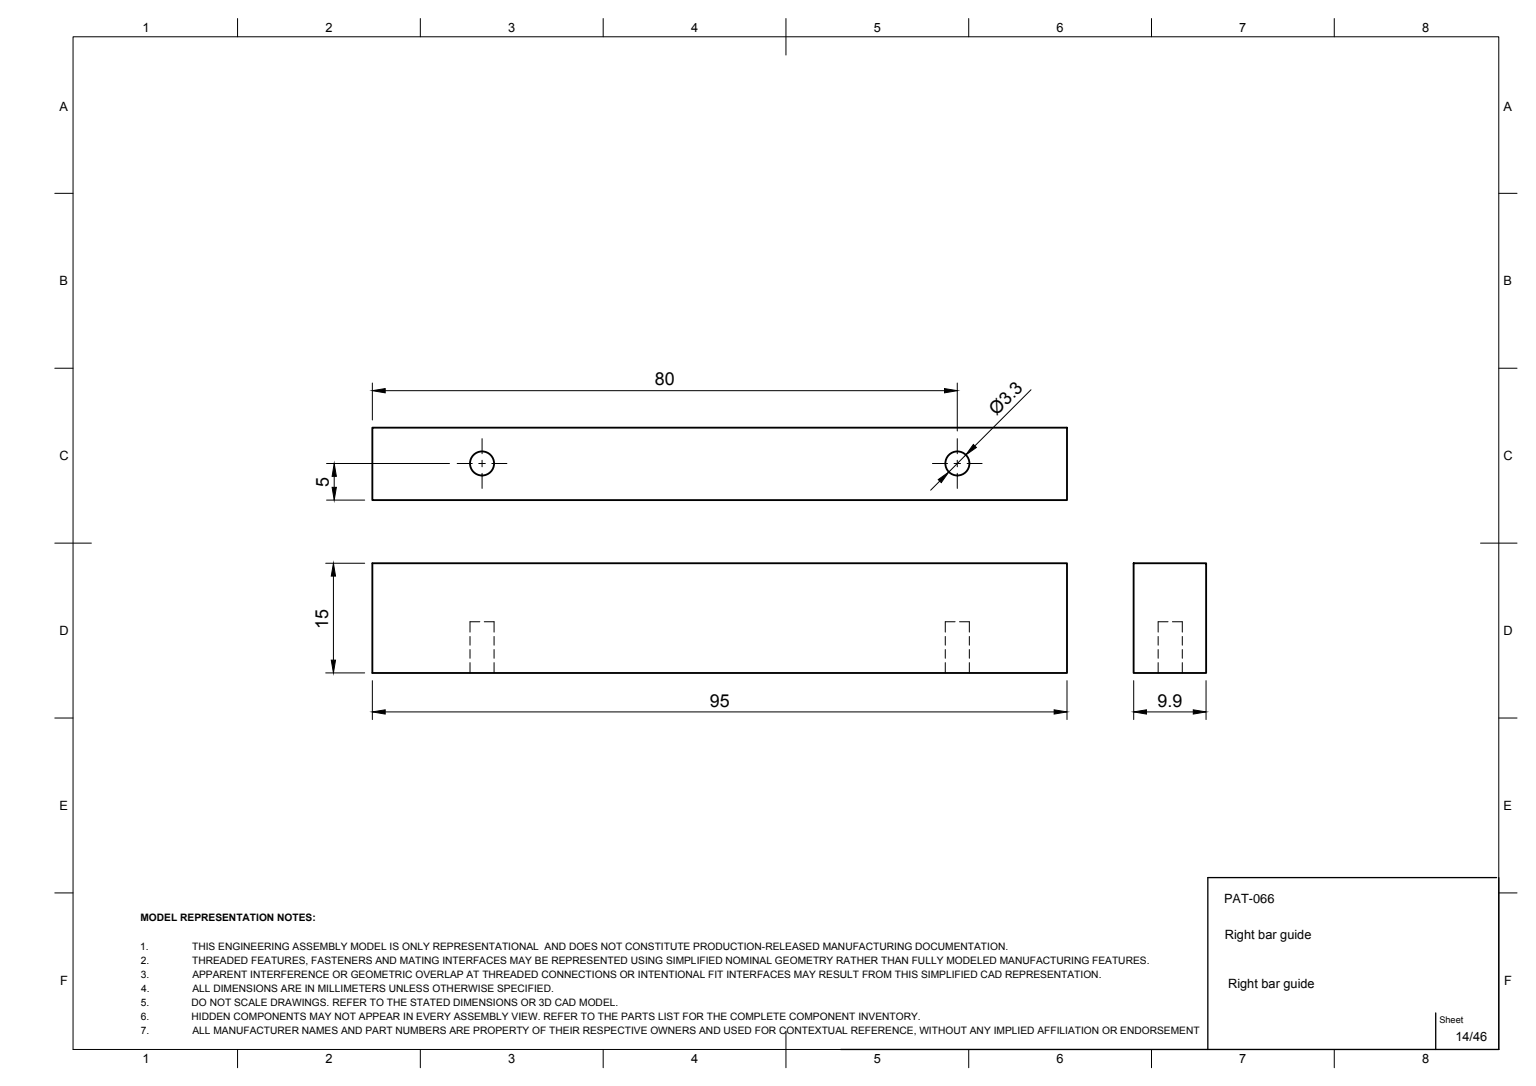
ISO-10303-21;
HEADER;
/* Generated by software containing ST-Developer
 * from STEP Tools, Inc. (www.steptools.com) 
 */

FILE_DESCRIPTION(
/* description */ ('Lever-operated bar clamp (toggle)'),
/* implementation_level */ '2;1');

FILE_NAME(
/* name */ 'Right bar guide.step',
/* time_stamp */ '2026-10-28T03:25:02-07:00',
/* author */ (''),
/* organization */ (''),
/* preprocessor_version */ 'ST-DEVELOPER v20.2',
/* originating_system */ 'Autodesk Translation Framework v15.17.0.0',
/* authorisation */ '');

FILE_SCHEMA (('AUTOMOTIVE_DESIGN { 1 0 10303 214 3 1 1 }'));
ENDSEC;

DATA;
#10=MECHANICAL_DESIGN_GEOMETRIC_PRESENTATION_REPRESENTATION('',(#419),#12413);
#343=SHAPE_REPRESENTATION_RELATIONSHIP('SRR','None',#12582,#381);
#381=ADVANCED_BREP_SHAPE_REPRESENTATION('',(#466),#12379);
#419=STYLED_ITEM('',(#12883),#466);
#466=MANIFOLD_SOLID_BREP('Body1',#6578);
#583=FACE_BOUND('',#1505,.T.);
#584=FACE_BOUND('',#1506,.T.);
#716=PLANE('',#7278);
#717=PLANE('',#7282);
#718=PLANE('',#7283);
#719=PLANE('',#7284);
#720=PLANE('',#7285);
#721=PLANE('',#7286);
#722=PLANE('',#7287);
#723=PLANE('',#7288);
#1006=FACE_OUTER_BOUND('',#1495,.T.);
#1007=FACE_OUTER_BOUND('',#1496,.T.);
#1008=FACE_OUTER_BOUND('',#1497,.T.);
#1009=FACE_OUTER_BOUND('',#1498,.T.);
#1010=FACE_OUTER_BOUND('',#1499,.T.);
#1011=FACE_OUTER_BOUND('',#1500,.T.);
#1012=FACE_OUTER_BOUND('',#1501,.T.);
#1013=FACE_OUTER_BOUND('',#1502,.T.);
#1014=FACE_OUTER_BOUND('',#1503,.T.);
#1015=FACE_OUTER_BOUND('',#1504,.T.);
#1495=EDGE_LOOP('',(#4931,#4932,#4933,#4934));
#1496=EDGE_LOOP('',(#4935));
#1497=EDGE_LOOP('',(#4936,#4937,#4938,#4939));
#1498=EDGE_LOOP('',(#4940));
#1499=EDGE_LOOP('',(#4941,#4942,#4943,#4944));
#1500=EDGE_LOOP('',(#4945,#4946,#4947,#4948));
#1501=EDGE_LOOP('',(#4949,#4950,#4951,#4952));
#1502=EDGE_LOOP('',(#4953,#4954,#4955,#4956));
#1503=EDGE_LOOP('',(#4957,#4958,#4959,#4960));
#1504=EDGE_LOOP('',(#4961,#4962,#4963,#4964));
#1505=EDGE_LOOP('',(#4965));
#1506=EDGE_LOOP('',(#4966));
#2000=LINE('',#10604,#2441);
#2001=LINE('',#10611,#2442);
#2002=LINE('',#10617,#2443);
#2003=LINE('',#10619,#2444);
#2004=LINE('',#10621,#2445);
#2005=LINE('',#10622,#2446);
#2006=LINE('',#10625,#2447);
#2007=LINE('',#10627,#2448);
#2008=LINE('',#10628,#2449);
#2009=LINE('',#10631,#2450);
#2010=LINE('',#10633,#2451);
#2011=LINE('',#10634,#2452);
#2012=LINE('',#10636,#2453);
#2013=LINE('',#10637,#2454);
#2441=VECTOR('',#8519,0.165);
#2442=VECTOR('',#8528,0.165);
#2443=VECTOR('',#8535,1.);
#2444=VECTOR('',#8536,1.);
#2445=VECTOR('',#8537,1.);
#2446=VECTOR('',#8538,1.);
#2447=VECTOR('',#8541,1.);
#2448=VECTOR('',#8542,1.);
#2449=VECTOR('',#8543,1.);
#2450=VECTOR('',#8546,1.);
#2451=VECTOR('',#8547,1.);
#2452=VECTOR('',#8548,1.);
#2453=VECTOR('',#8551,1.);
#2454=VECTOR('',#8552,1.);
#2839=CIRCLE('',#7276,0.165);
#2840=CIRCLE('',#7277,0.165);
#2841=CIRCLE('',#7280,0.165);
#2842=CIRCLE('',#7281,0.165);
#3244=VERTEX_POINT('',#10601);
#3245=VERTEX_POINT('',#10603);
#3246=VERTEX_POINT('',#10608);
#3247=VERTEX_POINT('',#10610);
#3248=VERTEX_POINT('',#10615);
#3249=VERTEX_POINT('',#10616);
#3250=VERTEX_POINT('',#10618);
#3251=VERTEX_POINT('',#10620);
#3252=VERTEX_POINT('',#10624);
#3253=VERTEX_POINT('',#10626);
#3254=VERTEX_POINT('',#10630);
#3255=VERTEX_POINT('',#10632);
#3870=EDGE_CURVE('',#3244,#3244,#2839,.T.);
#3871=EDGE_CURVE('',#3244,#3245,#2000,.T.);
#3872=EDGE_CURVE('',#3245,#3245,#2840,.T.);
#3873=EDGE_CURVE('',#3246,#3246,#2841,.T.);
#3874=EDGE_CURVE('',#3246,#3247,#2001,.T.);
#3875=EDGE_CURVE('',#3247,#3247,#2842,.T.);
#3876=EDGE_CURVE('',#3248,#3249,#2002,.T.);
#3877=EDGE_CURVE('',#3249,#3250,#2003,.T.);
#3878=EDGE_CURVE('',#3251,#3250,#2004,.T.);
#3879=EDGE_CURVE('',#3248,#3251,#2005,.T.);
#3880=EDGE_CURVE('',#3252,#3248,#2006,.T.);
#3881=EDGE_CURVE('',#3253,#3251,#2007,.T.);
#3882=EDGE_CURVE('',#3252,#3253,#2008,.T.);
#3883=EDGE_CURVE('',#3254,#3252,#2009,.T.);
#3884=EDGE_CURVE('',#3255,#3253,#2010,.T.);
#3885=EDGE_CURVE('',#3254,#3255,#2011,.T.);
#3886=EDGE_CURVE('',#3249,#3254,#2012,.T.);
#3887=EDGE_CURVE('',#3250,#3255,#2013,.T.);
#4931=ORIENTED_EDGE('',*,*,#3870,.F.);
#4932=ORIENTED_EDGE('',*,*,#3871,.T.);
#4933=ORIENTED_EDGE('',*,*,#3872,.T.);
#4934=ORIENTED_EDGE('',*,*,#3871,.F.);
#4935=ORIENTED_EDGE('',*,*,#3872,.F.);
#4936=ORIENTED_EDGE('',*,*,#3873,.F.);
#4937=ORIENTED_EDGE('',*,*,#3874,.T.);
#4938=ORIENTED_EDGE('',*,*,#3875,.T.);
#4939=ORIENTED_EDGE('',*,*,#3874,.F.);
#4940=ORIENTED_EDGE('',*,*,#3875,.F.);
#4941=ORIENTED_EDGE('',*,*,#3876,.T.);
#4942=ORIENTED_EDGE('',*,*,#3877,.T.);
#4943=ORIENTED_EDGE('',*,*,#3878,.F.);
#4944=ORIENTED_EDGE('',*,*,#3879,.F.);
#4945=ORIENTED_EDGE('',*,*,#3880,.T.);
#4946=ORIENTED_EDGE('',*,*,#3879,.T.);
#4947=ORIENTED_EDGE('',*,*,#3881,.F.);
#4948=ORIENTED_EDGE('',*,*,#3882,.F.);
#4949=ORIENTED_EDGE('',*,*,#3883,.T.);
#4950=ORIENTED_EDGE('',*,*,#3882,.T.);
#4951=ORIENTED_EDGE('',*,*,#3884,.F.);
#4952=ORIENTED_EDGE('',*,*,#3885,.F.);
#4953=ORIENTED_EDGE('',*,*,#3886,.T.);
#4954=ORIENTED_EDGE('',*,*,#3885,.T.);
#4955=ORIENTED_EDGE('',*,*,#3887,.F.);
#4956=ORIENTED_EDGE('',*,*,#3877,.F.);
#4957=ORIENTED_EDGE('',*,*,#3887,.T.);
#4958=ORIENTED_EDGE('',*,*,#3884,.T.);
#4959=ORIENTED_EDGE('',*,*,#3881,.T.);
#4960=ORIENTED_EDGE('',*,*,#3878,.T.);
#4961=ORIENTED_EDGE('',*,*,#3886,.F.);
#4962=ORIENTED_EDGE('',*,*,#3876,.F.);
#4963=ORIENTED_EDGE('',*,*,#3880,.F.);
#4964=ORIENTED_EDGE('',*,*,#3883,.F.);
#4965=ORIENTED_EDGE('',*,*,#3870,.T.);
#4966=ORIENTED_EDGE('',*,*,#3873,.T.);
#6086=CYLINDRICAL_SURFACE('',#7275,0.165);
#6087=CYLINDRICAL_SURFACE('',#7279,0.165);
#6281=ADVANCED_FACE('',(#1006),#6086,.F.);
#6282=ADVANCED_FACE('',(#1007),#716,.F.);
#6283=ADVANCED_FACE('',(#1008),#6087,.F.);
#6284=ADVANCED_FACE('',(#1009),#717,.F.);
#6285=ADVANCED_FACE('',(#1010),#718,.T.);
#6286=ADVANCED_FACE('',(#1011),#719,.T.);
#6287=ADVANCED_FACE('',(#1012),#720,.T.);
#6288=ADVANCED_FACE('',(#1013),#721,.T.);
#6289=ADVANCED_FACE('',(#1014),#722,.T.);
#6290=ADVANCED_FACE('',(#1015,#583,#584),#723,.F.);
#6578=CLOSED_SHELL('',(#6281,#6282,#6283,#6284,#6285,#6286,#6287,#6288,
#6289,#6290));
#7274=AXIS2_PLACEMENT_3D('',#10599,#8513,#8514);
#7275=AXIS2_PLACEMENT_3D('',#10600,#8515,#8516);
#7276=AXIS2_PLACEMENT_3D('',#10602,#8517,#8518);
#7277=AXIS2_PLACEMENT_3D('',#10605,#8520,#8521);
#7278=AXIS2_PLACEMENT_3D('',#10606,#8522,#8523);
#7279=AXIS2_PLACEMENT_3D('',#10607,#8524,#8525);
#7280=AXIS2_PLACEMENT_3D('',#10609,#8526,#8527);
#7281=AXIS2_PLACEMENT_3D('',#10612,#8529,#8530);
#7282=AXIS2_PLACEMENT_3D('',#10613,#8531,#8532);
#7283=AXIS2_PLACEMENT_3D('',#10614,#8533,#8534);
#7284=AXIS2_PLACEMENT_3D('',#10623,#8539,#8540);
#7285=AXIS2_PLACEMENT_3D('',#10629,#8544,#8545);
#7286=AXIS2_PLACEMENT_3D('',#10635,#8549,#8550);
#7287=AXIS2_PLACEMENT_3D('',#10638,#8553,#8554);
#7288=AXIS2_PLACEMENT_3D('',#10639,#8555,#8556);
#8513=DIRECTION('axis',(0.,0.,1.));
#8514=DIRECTION('refdir',(1.,0.,0.));
#8515=DIRECTION('center_axis',(0.,0.,1.));
#8516=DIRECTION('ref_axis',(1.,0.,0.));
#8517=DIRECTION('center_axis',(0.,0.,1.));
#8518=DIRECTION('ref_axis',(1.,0.,0.));
#8519=DIRECTION('',(0.,0.,1.));
#8520=DIRECTION('center_axis',(0.,0.,1.));
#8521=DIRECTION('ref_axis',(1.,0.,0.));
#8522=DIRECTION('center_axis',(0.,0.,1.));
#8523=DIRECTION('ref_axis',(1.,0.,0.));
#8524=DIRECTION('center_axis',(0.,0.,1.));
#8525=DIRECTION('ref_axis',(1.,0.,0.));
#8526=DIRECTION('center_axis',(0.,0.,1.));
#8527=DIRECTION('ref_axis',(1.,0.,0.));
#8528=DIRECTION('',(0.,0.,1.));
#8529=DIRECTION('center_axis',(0.,0.,1.));
#8530=DIRECTION('ref_axis',(1.,0.,0.));
#8531=DIRECTION('center_axis',(0.,0.,1.));
#8532=DIRECTION('ref_axis',(1.,0.,0.));
#8533=DIRECTION('center_axis',(0.,1.,0.));
#8534=DIRECTION('ref_axis',(-1.,0.,0.));
#8535=DIRECTION('',(-1.,0.,0.));
#8536=DIRECTION('',(0.,0.,1.));
#8537=DIRECTION('',(-1.,0.,0.));
#8538=DIRECTION('',(0.,0.,1.));
#8539=DIRECTION('center_axis',(1.,0.,0.));
#8540=DIRECTION('ref_axis',(0.,1.,0.));
#8541=DIRECTION('',(0.,1.,0.));
#8542=DIRECTION('',(0.,1.,0.));
#8543=DIRECTION('',(0.,0.,1.));
#8544=DIRECTION('center_axis',(0.,-1.,0.));
#8545=DIRECTION('ref_axis',(1.,0.,0.));
#8546=DIRECTION('',(1.,0.,0.));
#8547=DIRECTION('',(1.,0.,0.));
#8548=DIRECTION('',(0.,0.,1.));
#8549=DIRECTION('center_axis',(-1.,0.,0.));
#8550=DIRECTION('ref_axis',(0.,-1.,0.));
#8551=DIRECTION('',(0.,-1.,0.));
#8552=DIRECTION('',(0.,-1.,0.));
#8553=DIRECTION('center_axis',(0.,0.,1.));
#8554=DIRECTION('ref_axis',(1.,0.,0.));
#8555=DIRECTION('center_axis',(0.,0.,1.));
#8556=DIRECTION('ref_axis',(1.,0.,0.));
#10599=CARTESIAN_POINT('',(0.,0.,0.));
#10600=CARTESIAN_POINT('Origin',(1.5,-4.5,0.9));
#10601=CARTESIAN_POINT('',(1.335,-4.5,1.));
#10602=CARTESIAN_POINT('Origin',(1.5,-4.5,1.));
#10603=CARTESIAN_POINT('',(1.335,-4.5,1.7));
#10604=CARTESIAN_POINT('',(1.335,-4.5,0.9));
#10605=CARTESIAN_POINT('Origin',(1.5,-4.5,1.7));
#10606=CARTESIAN_POINT('Origin',(1.5,-4.5,1.7));
#10607=CARTESIAN_POINT('Origin',(1.5,2.,0.9));
#10608=CARTESIAN_POINT('',(1.335,2.,1.));
#10609=CARTESIAN_POINT('Origin',(1.5,2.,1.));
#10610=CARTESIAN_POINT('',(1.335,2.,1.7));
#10611=CARTESIAN_POINT('',(1.335,2.,0.9));
#10612=CARTESIAN_POINT('Origin',(1.5,2.,1.7));
#10613=CARTESIAN_POINT('Origin',(1.5,2.,1.7));
#10614=CARTESIAN_POINT('Origin',(2.,3.5,1.));
#10615=CARTESIAN_POINT('',(2.,3.5,1.));
#10616=CARTESIAN_POINT('',(1.01,3.5,1.));
#10617=CARTESIAN_POINT('',(2.,3.5,1.));
#10618=CARTESIAN_POINT('',(1.01,3.5,2.5));
#10619=CARTESIAN_POINT('',(1.01,3.5,1.));
#10620=CARTESIAN_POINT('',(2.,3.5,2.5));
#10621=CARTESIAN_POINT('',(2.,3.5,2.5));
#10622=CARTESIAN_POINT('',(2.,3.5,1.));
#10623=CARTESIAN_POINT('Origin',(2.,-6.,1.));
#10624=CARTESIAN_POINT('',(2.,-6.,1.));
#10625=CARTESIAN_POINT('',(2.,-6.,1.));
#10626=CARTESIAN_POINT('',(2.,-6.,2.5));
#10627=CARTESIAN_POINT('',(2.,-6.,2.5));
#10628=CARTESIAN_POINT('',(2.,-6.,1.));
#10629=CARTESIAN_POINT('Origin',(1.01,-6.,1.));
#10630=CARTESIAN_POINT('',(1.01,-6.,1.));
#10631=CARTESIAN_POINT('',(1.01,-6.,1.));
#10632=CARTESIAN_POINT('',(1.01,-6.,2.5));
#10633=CARTESIAN_POINT('',(1.01,-6.,2.5));
#10634=CARTESIAN_POINT('',(1.01,-6.,1.));
#10635=CARTESIAN_POINT('Origin',(1.01,3.5,1.));
#10636=CARTESIAN_POINT('',(1.01,3.5,1.));
#10637=CARTESIAN_POINT('',(1.01,3.5,2.5));
#10638=CARTESIAN_POINT('Origin',(1.505,-1.25,2.5));
#10639=CARTESIAN_POINT('Origin',(1.505,-1.25,1.));
#12333=UNCERTAINTY_MEASURE_WITH_UNIT(LENGTH_MEASURE(0.001),#12414,
'DISTANCE_ACCURACY_VALUE',
'Maximum model space distance between geometric entities at asserted c
onnectivities');
#12367=UNCERTAINTY_MEASURE_WITH_UNIT(LENGTH_MEASURE(0.001),#12414,
'DISTANCE_ACCURACY_VALUE',
'Maximum model space distance between geometric entities at asserted c
onnectivities');
#12379=(
GEOMETRIC_REPRESENTATION_CONTEXT(3)
GLOBAL_UNCERTAINTY_ASSIGNED_CONTEXT((#12333))
GLOBAL_UNIT_ASSIGNED_CONTEXT((#12414,#12416,#12417))
REPRESENTATION_CONTEXT('','3D')
);
#12413=(
GEOMETRIC_REPRESENTATION_CONTEXT(3)
GLOBAL_UNCERTAINTY_ASSIGNED_CONTEXT((#12367))
GLOBAL_UNIT_ASSIGNED_CONTEXT((#12414,#12416,#12417))
REPRESENTATION_CONTEXT('','3D')
);
#12414=(
LENGTH_UNIT()
NAMED_UNIT(*)
SI_UNIT(.CENTI.,.METRE.)
);
#12416=(
NAMED_UNIT(*)
PLANE_ANGLE_UNIT()
SI_UNIT($,.RADIAN.)
);
#12417=(
NAMED_UNIT(*)
SI_UNIT($,.STERADIAN.)
SOLID_ANGLE_UNIT()
);
#12429=SHAPE_DEFINITION_REPRESENTATION(#12474,#12582);
#12474=PRODUCT_DEFINITION_SHAPE('',$,#12628);
#12582=SHAPE_REPRESENTATION('',(#7274),#12379);
#12616=PRODUCT_DEFINITION_CONTEXT('part definition',#12753,'design');
#12628=PRODUCT_DEFINITION('Right bar guide','Right bar guide',#12673,#12616);
#12673=PRODUCT_DEFINITION_FORMATION('',$,#12766);
#12753=APPLICATION_CONTEXT(
'Core Data for Automotive Mechanical Design Process');
#12754=PRODUCT_CONTEXT('part definition',#12753,'mechanical');
#12766=PRODUCT('Right bar guide','Right bar guide','Right bar guide',(#12754));
#12877=COLOUR_RGB('Off White',0.89,0.88,0.83);
#12878=FILL_AREA_STYLE_COLOUR('',#12877);
#12879=FILL_AREA_STYLE('',(#12878));
#12880=SURFACE_STYLE_FILL_AREA(#12879);
#12881=SURFACE_SIDE_STYLE('',(#12880));
#12882=SURFACE_STYLE_USAGE(.BOTH.,#12881);
#12883=PRESENTATION_STYLE_ASSIGNMENT((#12882));
ENDSEC;
END-ISO-10303-21;
